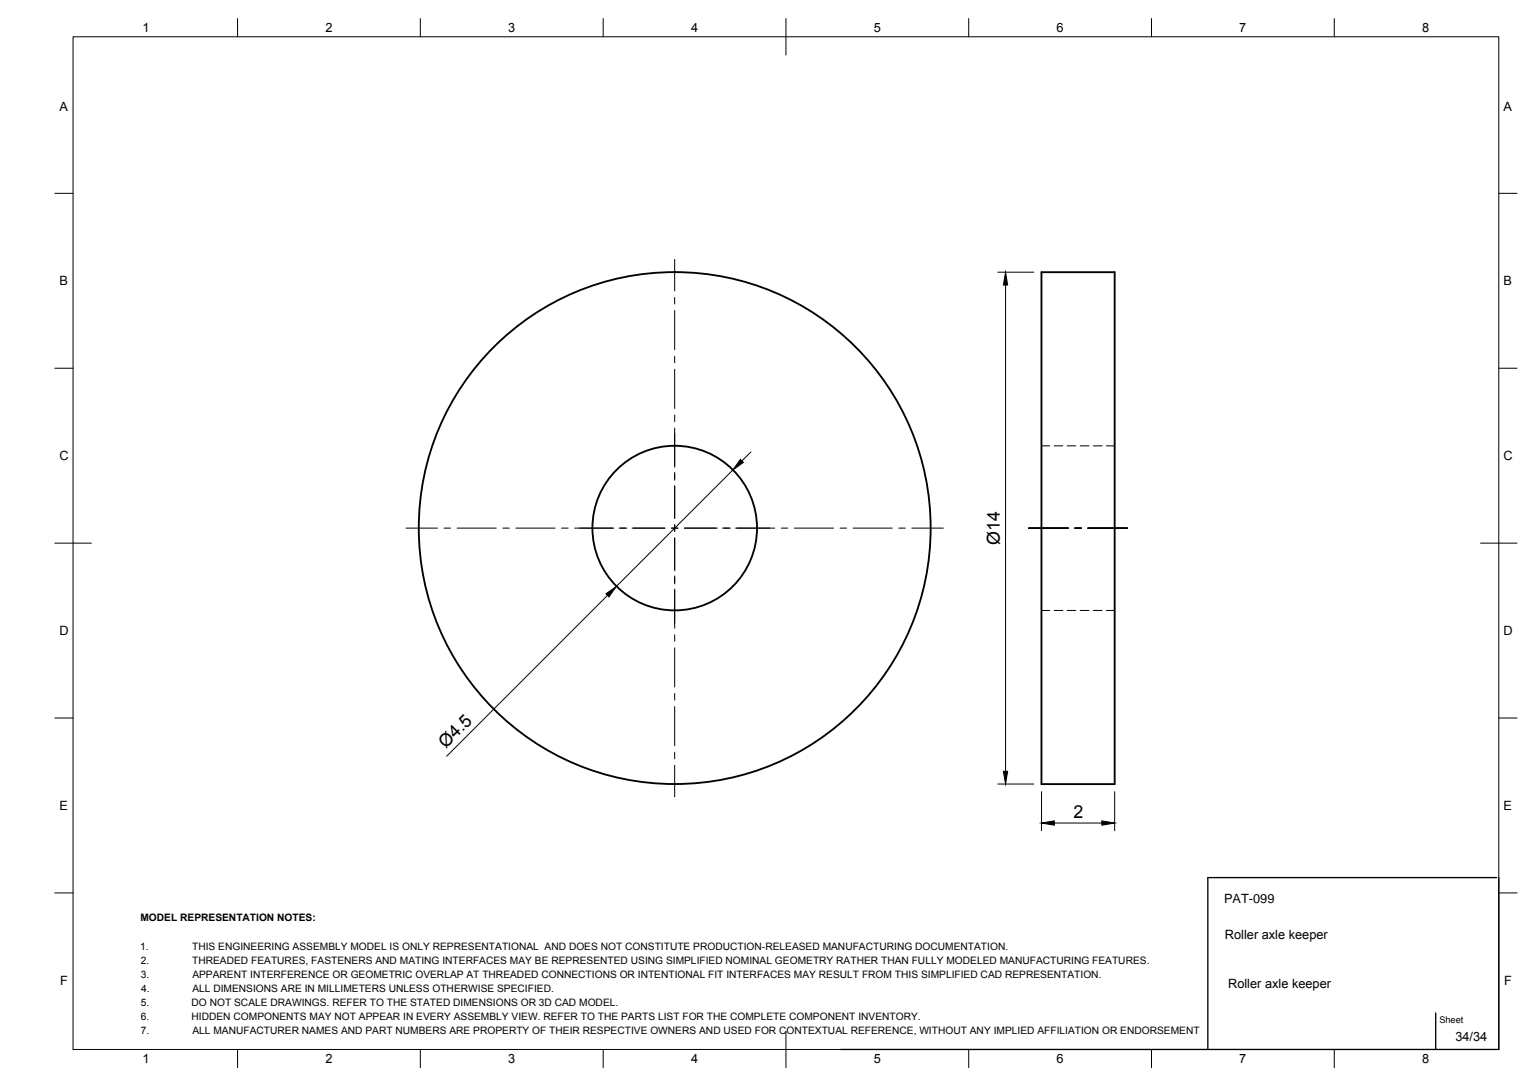
ISO-10303-21;
HEADER;
/* Generated by software containing ST-Developer
 * from STEP Tools, Inc. (www.steptools.com) 
 */

FILE_DESCRIPTION(
/* description */ ('PAT-099'),
/* implementation_level */ '2;1');

FILE_NAME(
/* name */ 'Roller axle keeper.step',
/* time_stamp */ '2026-10-29T17:25:42-07:00',
/* author */ (''),
/* organization */ (''),
/* preprocessor_version */ 'ST-DEVELOPER v20.2',
/* originating_system */ 'Autodesk Translation Framework v15.17.0.0',
/* authorisation */ '');

FILE_SCHEMA (('AUTOMOTIVE_DESIGN { 1 0 10303 214 3 1 1 }'));
ENDSEC;

DATA;
#10=MECHANICAL_DESIGN_GEOMETRIC_PRESENTATION_REPRESENTATION('',(#355),#11035);
#305=SHAPE_REPRESENTATION_RELATIONSHIP('SRR','None',#11176,#330);
#330=ADVANCED_BREP_SHAPE_REPRESENTATION('',(#387),#11026);
#355=STYLED_ITEM('',(#11386),#387);
#387=MANIFOLD_SOLID_BREP('Body1',#4724);
#511=FACE_BOUND('',#1263,.T.);
#512=FACE_BOUND('',#1265,.T.);
#629=PLANE('',#5469);
#630=PLANE('',#5470);
#869=FACE_OUTER_BOUND('',#1260,.T.);
#870=FACE_OUTER_BOUND('',#1261,.T.);
#871=FACE_OUTER_BOUND('',#1262,.T.);
#872=FACE_OUTER_BOUND('',#1264,.T.);
#1260=EDGE_LOOP('',(#4025,#4026,#4027,#4028));
#1261=EDGE_LOOP('',(#4029,#4030,#4031,#4032));
#1262=EDGE_LOOP('',(#4033));
#1263=EDGE_LOOP('',(#4034));
#1264=EDGE_LOOP('',(#4035));
#1265=EDGE_LOOP('',(#4036));
#1554=LINE('',#10269,#1806);
#1555=LINE('',#10275,#1807);
#1806=VECTOR('',#6777,0.225);
#1807=VECTOR('',#6784,0.7);
#2055=CIRCLE('',#5464,0.225);
#2056=CIRCLE('',#5465,0.225);
#2057=CIRCLE('',#5467,0.7);
#2058=CIRCLE('',#5468,0.7);
#2439=VERTEX_POINT('',#10266);
#2440=VERTEX_POINT('',#10268);
#2441=VERTEX_POINT('',#10272);
#2442=VERTEX_POINT('',#10274);
#2989=EDGE_CURVE('',#2439,#2439,#2055,.T.);
#2990=EDGE_CURVE('',#2439,#2440,#1554,.T.);
#2991=EDGE_CURVE('',#2440,#2440,#2056,.T.);
#2992=EDGE_CURVE('',#2441,#2441,#2057,.T.);
#2993=EDGE_CURVE('',#2441,#2442,#1555,.T.);
#2994=EDGE_CURVE('',#2442,#2442,#2058,.T.);
#4025=ORIENTED_EDGE('',*,*,#2989,.F.);
#4026=ORIENTED_EDGE('',*,*,#2990,.T.);
#4027=ORIENTED_EDGE('',*,*,#2991,.T.);
#4028=ORIENTED_EDGE('',*,*,#2990,.F.);
#4029=ORIENTED_EDGE('',*,*,#2992,.F.);
#4030=ORIENTED_EDGE('',*,*,#2993,.T.);
#4031=ORIENTED_EDGE('',*,*,#2994,.T.);
#4032=ORIENTED_EDGE('',*,*,#2993,.F.);
#4033=ORIENTED_EDGE('',*,*,#2992,.T.);
#4034=ORIENTED_EDGE('',*,*,#2989,.T.);
#4035=ORIENTED_EDGE('',*,*,#2994,.F.);
#4036=ORIENTED_EDGE('',*,*,#2991,.F.);
#4408=CYLINDRICAL_SURFACE('',#5463,0.225);
#4409=CYLINDRICAL_SURFACE('',#5466,0.7);
#4634=ADVANCED_FACE('',(#869),#4408,.F.);
#4635=ADVANCED_FACE('',(#870),#4409,.T.);
#4636=ADVANCED_FACE('',(#871,#511),#629,.T.);
#4637=ADVANCED_FACE('',(#872,#512),#630,.F.);
#4724=CLOSED_SHELL('',(#4634,#4635,#4636,#4637));
#5462=AXIS2_PLACEMENT_3D('',#10264,#6771,#6772);
#5463=AXIS2_PLACEMENT_3D('',#10265,#6773,#6774);
#5464=AXIS2_PLACEMENT_3D('',#10267,#6775,#6776);
#5465=AXIS2_PLACEMENT_3D('',#10270,#6778,#6779);
#5466=AXIS2_PLACEMENT_3D('',#10271,#6780,#6781);
#5467=AXIS2_PLACEMENT_3D('',#10273,#6782,#6783);
#5468=AXIS2_PLACEMENT_3D('',#10276,#6785,#6786);
#5469=AXIS2_PLACEMENT_3D('',#10277,#6787,#6788);
#5470=AXIS2_PLACEMENT_3D('',#10278,#6789,#6790);
#6771=DIRECTION('axis',(0.,0.,1.));
#6772=DIRECTION('refdir',(1.,0.,0.));
#6773=DIRECTION('center_axis',(0.,0.,1.));
#6774=DIRECTION('ref_axis',(1.,0.,0.));
#6775=DIRECTION('center_axis',(0.,0.,-1.));
#6776=DIRECTION('ref_axis',(1.,0.,0.));
#6777=DIRECTION('',(0.,0.,-1.));
#6778=DIRECTION('center_axis',(0.,0.,-1.));
#6779=DIRECTION('ref_axis',(1.,0.,0.));
#6780=DIRECTION('center_axis',(0.,0.,1.));
#6781=DIRECTION('ref_axis',(1.,0.,0.));
#6782=DIRECTION('center_axis',(0.,0.,1.));
#6783=DIRECTION('ref_axis',(1.,0.,0.));
#6784=DIRECTION('',(0.,0.,-1.));
#6785=DIRECTION('center_axis',(0.,0.,1.));
#6786=DIRECTION('ref_axis',(1.,0.,0.));
#6787=DIRECTION('center_axis',(0.,0.,1.));
#6788=DIRECTION('ref_axis',(1.,0.,0.));
#6789=DIRECTION('center_axis',(0.,0.,1.));
#6790=DIRECTION('ref_axis',(1.,0.,0.));
#10264=CARTESIAN_POINT('',(0.,0.,0.));
#10265=CARTESIAN_POINT('Origin',(4.,0.,6.3));
#10266=CARTESIAN_POINT('',(3.775,-2.75545529808154E-17,6.5));
#10267=CARTESIAN_POINT('Origin',(4.,0.,6.5));
#10268=CARTESIAN_POINT('',(3.775,-2.75545529808154E-17,6.3));
#10269=CARTESIAN_POINT('',(3.775,-2.75545529808154E-17,6.3));
#10270=CARTESIAN_POINT('Origin',(4.,0.,6.3));
#10271=CARTESIAN_POINT('Origin',(4.,0.,6.3));
#10272=CARTESIAN_POINT('',(3.3,-8.57252759403147E-17,6.5));
#10273=CARTESIAN_POINT('Origin',(4.,0.,6.5));
#10274=CARTESIAN_POINT('',(3.3,-8.57252759403147E-17,6.3));
#10275=CARTESIAN_POINT('',(3.3,-8.57252759403147E-17,6.3));
#10276=CARTESIAN_POINT('Origin',(4.,0.,6.3));
#10277=CARTESIAN_POINT('Origin',(4.,0.,6.5));
#10278=CARTESIAN_POINT('Origin',(4.,0.,6.3));
#10993=UNCERTAINTY_MEASURE_WITH_UNIT(LENGTH_MEASURE(0.001),#11036,
'DISTANCE_ACCURACY_VALUE',
'Maximum model space distance between geometric entities at asserted c
onnectivities');
#11002=UNCERTAINTY_MEASURE_WITH_UNIT(LENGTH_MEASURE(0.001),#11036,
'DISTANCE_ACCURACY_VALUE',
'Maximum model space distance between geometric entities at asserted c
onnectivities');
#11026=(
GEOMETRIC_REPRESENTATION_CONTEXT(3)
GLOBAL_UNCERTAINTY_ASSIGNED_CONTEXT((#10993))
GLOBAL_UNIT_ASSIGNED_CONTEXT((#11036,#11038,#11039))
REPRESENTATION_CONTEXT('','3D')
);
#11035=(
GEOMETRIC_REPRESENTATION_CONTEXT(3)
GLOBAL_UNCERTAINTY_ASSIGNED_CONTEXT((#11002))
GLOBAL_UNIT_ASSIGNED_CONTEXT((#11036,#11038,#11039))
REPRESENTATION_CONTEXT('','3D')
);
#11036=(
LENGTH_UNIT()
NAMED_UNIT(*)
SI_UNIT(.CENTI.,.METRE.)
);
#11038=(
NAMED_UNIT(*)
PLANE_ANGLE_UNIT()
SI_UNIT($,.RADIAN.)
);
#11039=(
NAMED_UNIT(*)
SI_UNIT($,.STERADIAN.)
SOLID_ANGLE_UNIT()
);
#11063=SHAPE_DEFINITION_REPRESENTATION(#11101,#11176);
#11101=PRODUCT_DEFINITION_SHAPE('',$,#11209);
#11176=SHAPE_REPRESENTATION('',(#5462),#11026);
#11185=PRODUCT_DEFINITION_CONTEXT('part definition',#11283,'design');
#11209=PRODUCT_DEFINITION('Roller axle keeper','Roller axle keeper',#11241,
#11185);
#11241=PRODUCT_DEFINITION_FORMATION('',$,#11308);
#11283=APPLICATION_CONTEXT(
'Core Data for Automotive Mechanical Design Process');
#11284=PRODUCT_CONTEXT('part definition',#11283,'mechanical');
#11308=PRODUCT('Roller axle keeper','Roller axle keeper',
'Roller axle keeper',(#11284));
#11380=COLOUR_RGB('Grey',0.48,0.52,0.57);
#11381=FILL_AREA_STYLE_COLOUR('',#11380);
#11382=FILL_AREA_STYLE('',(#11381));
#11383=SURFACE_STYLE_FILL_AREA(#11382);
#11384=SURFACE_SIDE_STYLE('',(#11383));
#11385=SURFACE_STYLE_USAGE(.BOTH.,#11384);
#11386=PRESENTATION_STYLE_ASSIGNMENT((#11385));
ENDSEC;
END-ISO-10303-21;
